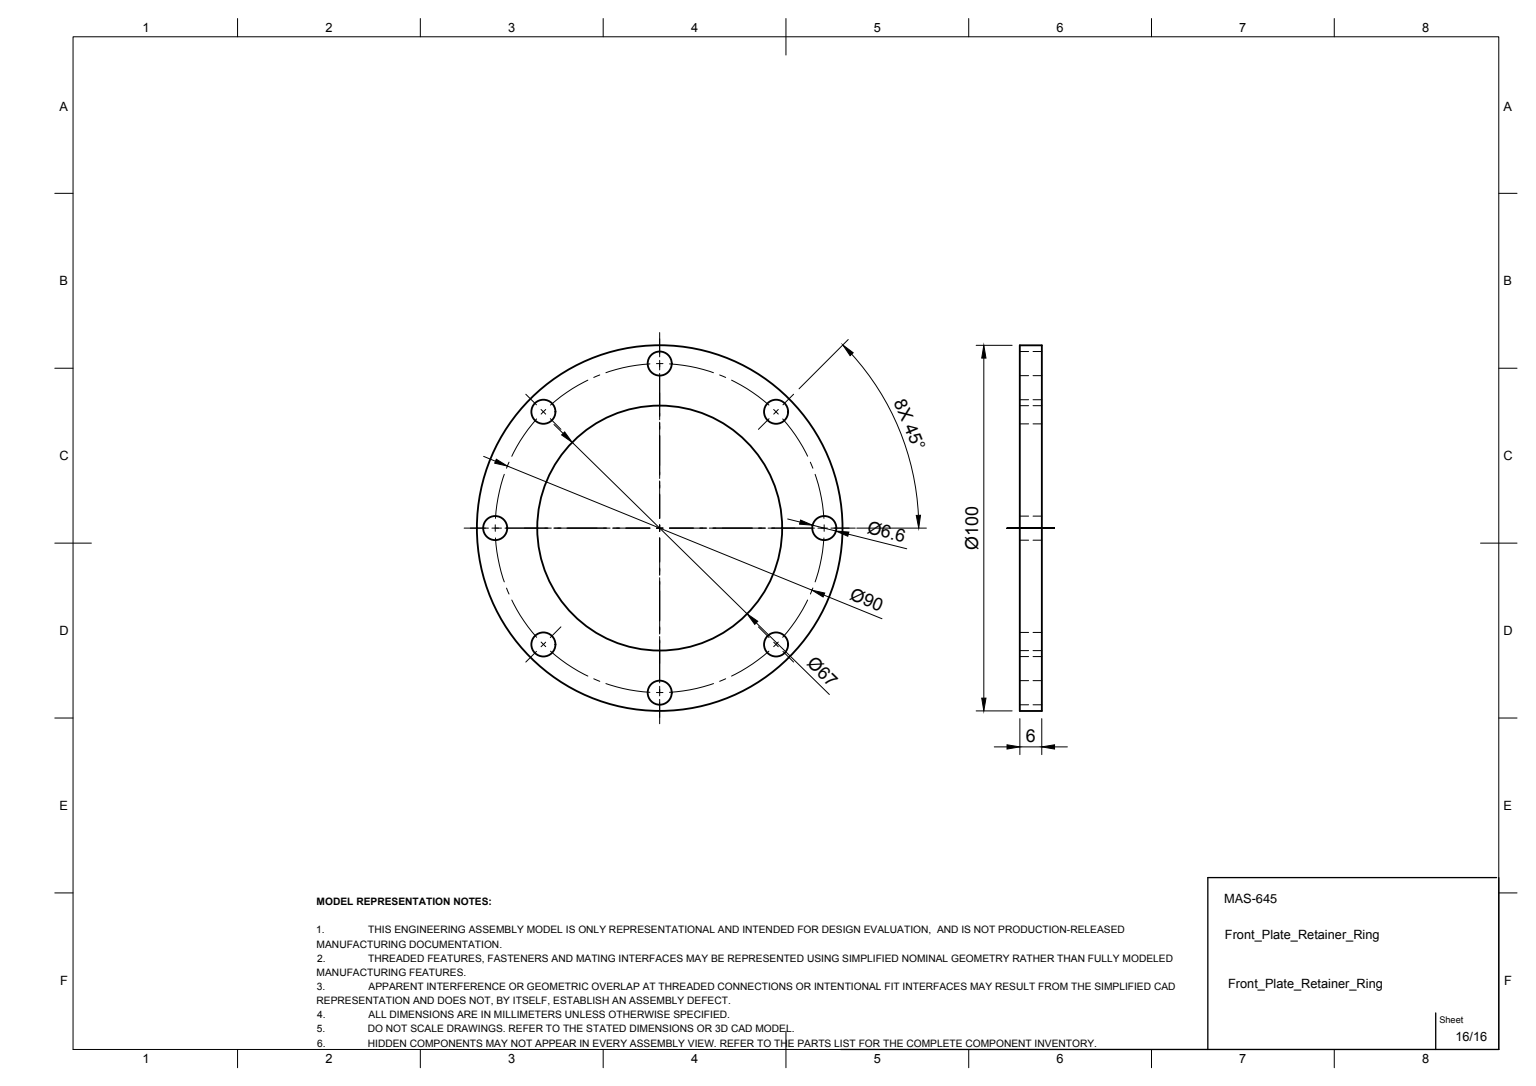
ISO-10303-21;
HEADER;
FILE_DESCRIPTION((''),'2;1');
FILE_NAME('Front_Plate_Retainer_Ring.step','2026-10-09T10:54:55-07:00',(''),(''),'','','');
FILE_SCHEMA (('AUTOMOTIVE_DESIGN { 1 0 10303 214 3 1 1 }'));
ENDSEC;
DATA;
#10=MECHANICAL_DESIGN_GEOMETRIC_PRESENTATION_REPRESENTATION('',(#609),#63824);
#579=SHAPE_REPRESENTATION_RELATIONSHIP('SRR','None',#63893,#594) ;
#594=ADVANCED_BREP_SHAPE_REPRESENTATION('',(#624),#63823) ;
#609=STYLED_ITEM('',(#63963),#624) ;
#624=MANIFOLD_SOLID_BREP('Body1',#15508) ;
#814=FACE_BOUND('',#3455,.T.) ;
#815=FACE_BOUND('',#3456,.T.) ;
#816=FACE_BOUND('',#3457,.T.) ;
#817=FACE_BOUND('',#3458,.T.) ;
#818=FACE_BOUND('',#3459,.T.) ;
#819=FACE_BOUND('',#3460,.T.) ;
#820=FACE_BOUND('',#3461,.T.) ;
#821=FACE_BOUND('',#3462,.T.) ;
#822=FACE_BOUND('',#3463,.T.) ;
#823=FACE_BOUND('',#3465,.T.) ;
#824=FACE_BOUND('',#3466,.T.) ;
#825=FACE_BOUND('',#3467,.T.) ;
#826=FACE_BOUND('',#3468,.T.) ;
#827=FACE_BOUND('',#3469,.T.) ;
#828=FACE_BOUND('',#3470,.T.) ;
#829=FACE_BOUND('',#3471,.T.) ;
#830=FACE_BOUND('',#3472,.T.) ;
#831=FACE_BOUND('',#3473,.T.) ;
#1114=PLANE('',#17883) ;
#1115=PLANE('',#17884) ;
#1535=CYLINDRICAL_SURFACE('',#17853,3.3) ;
#1536=CYLINDRICAL_SURFACE('',#17856,3.3) ;
#1537=CYLINDRICAL_SURFACE('',#17859,3.3) ;
#1538=CYLINDRICAL_SURFACE('',#17862,3.3) ;
#1539=CYLINDRICAL_SURFACE('',#17865,3.3) ;
#1540=CYLINDRICAL_SURFACE('',#17868,3.3) ;
#1541=CYLINDRICAL_SURFACE('',#17871,3.3) ;
#1542=CYLINDRICAL_SURFACE('',#17874,3.3) ;
#1543=CYLINDRICAL_SURFACE('',#17877,33.5) ;
#1544=CYLINDRICAL_SURFACE('',#17880,50.) ;
#2394=FACE_OUTER_BOUND('',#3444,.T.) ;
#2395=FACE_OUTER_BOUND('',#3445,.T.) ;
#2396=FACE_OUTER_BOUND('',#3446,.T.) ;
#2397=FACE_OUTER_BOUND('',#3447,.T.) ;
#2398=FACE_OUTER_BOUND('',#3448,.T.) ;
#2399=FACE_OUTER_BOUND('',#3449,.T.) ;
#2400=FACE_OUTER_BOUND('',#3450,.T.) ;
#2401=FACE_OUTER_BOUND('',#3451,.T.) ;
#2402=FACE_OUTER_BOUND('',#3452,.T.) ;
#2403=FACE_OUTER_BOUND('',#3453,.T.) ;
#2404=FACE_OUTER_BOUND('',#3454,.T.) ;
#2405=FACE_OUTER_BOUND('',#3464,.T.) ;
#3444=EDGE_LOOP('',(#14436,#14437,#14438,#14439)) ;
#3445=EDGE_LOOP('',(#14440,#14441,#14442,#14443)) ;
#3446=EDGE_LOOP('',(#14444,#14445,#14446,#14447)) ;
#3447=EDGE_LOOP('',(#14448,#14449,#14450,#14451)) ;
#3448=EDGE_LOOP('',(#14452,#14453,#14454,#14455)) ;
#3449=EDGE_LOOP('',(#14456,#14457,#14458,#14459)) ;
#3450=EDGE_LOOP('',(#14460,#14461,#14462,#14463)) ;
#3451=EDGE_LOOP('',(#14464,#14465,#14466,#14467)) ;
#3452=EDGE_LOOP('',(#14468,#14469,#14470,#14471)) ;
#3453=EDGE_LOOP('',(#14472,#14473,#14474,#14475)) ;
#3454=EDGE_LOOP('',(#14476)) ;
#3455=EDGE_LOOP('',(#14477)) ;
#3456=EDGE_LOOP('',(#14478)) ;
#3457=EDGE_LOOP('',(#14479)) ;
#3458=EDGE_LOOP('',(#14480)) ;
#3459=EDGE_LOOP('',(#14481)) ;
#3460=EDGE_LOOP('',(#14482)) ;
#3461=EDGE_LOOP('',(#14483)) ;
#3462=EDGE_LOOP('',(#14484)) ;
#3463=EDGE_LOOP('',(#14485)) ;
#3464=EDGE_LOOP('',(#14486)) ;
#3465=EDGE_LOOP('',(#14487)) ;
#3466=EDGE_LOOP('',(#14488)) ;
#3467=EDGE_LOOP('',(#14489)) ;
#3468=EDGE_LOOP('',(#14490)) ;
#3469=EDGE_LOOP('',(#14491)) ;
#3470=EDGE_LOOP('',(#14492)) ;
#3471=EDGE_LOOP('',(#14493)) ;
#3472=EDGE_LOOP('',(#14494)) ;
#3473=EDGE_LOOP('',(#14495)) ;
#4670=CIRCLE('',#17854,3.3) ;
#4671=CIRCLE('',#17855,3.3) ;
#4672=CIRCLE('',#17857,3.3) ;
#4673=CIRCLE('',#17858,3.3) ;
#4674=CIRCLE('',#17860,3.3) ;
#4675=CIRCLE('',#17861,3.3) ;
#4676=CIRCLE('',#17863,3.3) ;
#4677=CIRCLE('',#17864,3.3) ;
#4678=CIRCLE('',#17866,3.3) ;
#4679=CIRCLE('',#17867,3.3) ;
#4680=CIRCLE('',#17869,3.3) ;
#4681=CIRCLE('',#17870,3.3) ;
#4682=CIRCLE('',#17872,3.3) ;
#4683=CIRCLE('',#17873,3.3) ;
#4684=CIRCLE('',#17875,3.3) ;
#4685=CIRCLE('',#17876,3.3) ;
#4686=CIRCLE('',#17878,33.5) ;
#4687=CIRCLE('',#17879,33.5) ;
#4688=CIRCLE('',#17881,50.) ;
#4689=CIRCLE('',#17882,50.) ;
#5336=LINE('',#63716,#5992) ;
#5337=LINE('',#63722,#5993) ;
#5338=LINE('',#63728,#5994) ;
#5339=LINE('',#63734,#5995) ;
#5340=LINE('',#63740,#5996) ;
#5341=LINE('',#63746,#5997) ;
#5342=LINE('',#63752,#5998) ;
#5343=LINE('',#63758,#5999) ;
#5344=LINE('',#63764,#6000) ;
#5345=LINE('',#63770,#6001) ;
#5992=VECTOR('',#22908,3.3) ;
#5993=VECTOR('',#22915,3.3) ;
#5994=VECTOR('',#22922,3.3) ;
#5995=VECTOR('',#22929,3.3) ;
#5996=VECTOR('',#22936,3.3) ;
#5997=VECTOR('',#22943,3.3) ;
#5998=VECTOR('',#22950,3.3) ;
#5999=VECTOR('',#22957,3.3) ;
#6000=VECTOR('',#22964,33.5) ;
#6001=VECTOR('',#22971,50.) ;
#7435=VERTEX_POINT('',#63713) ;
#7436=VERTEX_POINT('',#63715) ;
#7437=VERTEX_POINT('',#63719) ;
#7438=VERTEX_POINT('',#63721) ;
#7439=VERTEX_POINT('',#63725) ;
#7440=VERTEX_POINT('',#63727) ;
#7441=VERTEX_POINT('',#63731) ;
#7442=VERTEX_POINT('',#63733) ;
#7443=VERTEX_POINT('',#63737) ;
#7444=VERTEX_POINT('',#63739) ;
#7445=VERTEX_POINT('',#63743) ;
#7446=VERTEX_POINT('',#63745) ;
#7447=VERTEX_POINT('',#63749) ;
#7448=VERTEX_POINT('',#63751) ;
#7449=VERTEX_POINT('',#63755) ;
#7450=VERTEX_POINT('',#63757) ;
#7451=VERTEX_POINT('',#63761) ;
#7452=VERTEX_POINT('',#63763) ;
#7453=VERTEX_POINT('',#63767) ;
#7454=VERTEX_POINT('',#63769) ;
#9772=EDGE_CURVE('',#7435,#7435,#4670,.T.) ;
#9773=EDGE_CURVE('',#7435,#7436,#5336,.T.) ;
#9774=EDGE_CURVE('',#7436,#7436,#4671,.T.) ;
#9775=EDGE_CURVE('',#7437,#7437,#4672,.T.) ;
#9776=EDGE_CURVE('',#7437,#7438,#5337,.T.) ;
#9777=EDGE_CURVE('',#7438,#7438,#4673,.T.) ;
#9778=EDGE_CURVE('',#7439,#7439,#4674,.T.) ;
#9779=EDGE_CURVE('',#7439,#7440,#5338,.T.) ;
#9780=EDGE_CURVE('',#7440,#7440,#4675,.T.) ;
#9781=EDGE_CURVE('',#7441,#7441,#4676,.T.) ;
#9782=EDGE_CURVE('',#7441,#7442,#5339,.T.) ;
#9783=EDGE_CURVE('',#7442,#7442,#4677,.T.) ;
#9784=EDGE_CURVE('',#7443,#7443,#4678,.T.) ;
#9785=EDGE_CURVE('',#7443,#7444,#5340,.T.) ;
#9786=EDGE_CURVE('',#7444,#7444,#4679,.T.) ;
#9787=EDGE_CURVE('',#7445,#7445,#4680,.T.) ;
#9788=EDGE_CURVE('',#7445,#7446,#5341,.T.) ;
#9789=EDGE_CURVE('',#7446,#7446,#4681,.T.) ;
#9790=EDGE_CURVE('',#7447,#7447,#4682,.T.) ;
#9791=EDGE_CURVE('',#7447,#7448,#5342,.T.) ;
#9792=EDGE_CURVE('',#7448,#7448,#4683,.T.) ;
#9793=EDGE_CURVE('',#7449,#7449,#4684,.T.) ;
#9794=EDGE_CURVE('',#7449,#7450,#5343,.T.) ;
#9795=EDGE_CURVE('',#7450,#7450,#4685,.T.) ;
#9796=EDGE_CURVE('',#7451,#7451,#4686,.T.) ;
#9797=EDGE_CURVE('',#7451,#7452,#5344,.T.) ;
#9798=EDGE_CURVE('',#7452,#7452,#4687,.T.) ;
#9799=EDGE_CURVE('',#7453,#7453,#4688,.T.) ;
#9800=EDGE_CURVE('',#7453,#7454,#5345,.T.) ;
#9801=EDGE_CURVE('',#7454,#7454,#4689,.T.) ;
#14436=ORIENTED_EDGE('',*,*,#9772,.T.) ;
#14437=ORIENTED_EDGE('',*,*,#9773,.T.) ;
#14438=ORIENTED_EDGE('',*,*,#9774,.T.) ;
#14439=ORIENTED_EDGE('',*,*,#9773,.F.) ;
#14440=ORIENTED_EDGE('',*,*,#9775,.T.) ;
#14441=ORIENTED_EDGE('',*,*,#9776,.T.) ;
#14442=ORIENTED_EDGE('',*,*,#9777,.T.) ;
#14443=ORIENTED_EDGE('',*,*,#9776,.F.) ;
#14444=ORIENTED_EDGE('',*,*,#9778,.T.) ;
#14445=ORIENTED_EDGE('',*,*,#9779,.T.) ;
#14446=ORIENTED_EDGE('',*,*,#9780,.T.) ;
#14447=ORIENTED_EDGE('',*,*,#9779,.F.) ;
#14448=ORIENTED_EDGE('',*,*,#9781,.T.) ;
#14449=ORIENTED_EDGE('',*,*,#9782,.T.) ;
#14450=ORIENTED_EDGE('',*,*,#9783,.T.) ;
#14451=ORIENTED_EDGE('',*,*,#9782,.F.) ;
#14452=ORIENTED_EDGE('',*,*,#9784,.T.) ;
#14453=ORIENTED_EDGE('',*,*,#9785,.T.) ;
#14454=ORIENTED_EDGE('',*,*,#9786,.T.) ;
#14455=ORIENTED_EDGE('',*,*,#9785,.F.) ;
#14456=ORIENTED_EDGE('',*,*,#9787,.T.) ;
#14457=ORIENTED_EDGE('',*,*,#9788,.T.) ;
#14458=ORIENTED_EDGE('',*,*,#9789,.T.) ;
#14459=ORIENTED_EDGE('',*,*,#9788,.F.) ;
#14460=ORIENTED_EDGE('',*,*,#9790,.T.) ;
#14461=ORIENTED_EDGE('',*,*,#9791,.T.) ;
#14462=ORIENTED_EDGE('',*,*,#9792,.T.) ;
#14463=ORIENTED_EDGE('',*,*,#9791,.F.) ;
#14464=ORIENTED_EDGE('',*,*,#9793,.T.) ;
#14465=ORIENTED_EDGE('',*,*,#9794,.T.) ;
#14466=ORIENTED_EDGE('',*,*,#9795,.T.) ;
#14467=ORIENTED_EDGE('',*,*,#9794,.F.) ;
#14468=ORIENTED_EDGE('',*,*,#9796,.T.) ;
#14469=ORIENTED_EDGE('',*,*,#9797,.T.) ;
#14470=ORIENTED_EDGE('',*,*,#9798,.T.) ;
#14471=ORIENTED_EDGE('',*,*,#9797,.F.) ;
#14472=ORIENTED_EDGE('',*,*,#9799,.T.) ;
#14473=ORIENTED_EDGE('',*,*,#9800,.T.) ;
#14474=ORIENTED_EDGE('',*,*,#9801,.T.) ;
#14475=ORIENTED_EDGE('',*,*,#9800,.F.) ;
#14476=ORIENTED_EDGE('',*,*,#9799,.F.) ;
#14477=ORIENTED_EDGE('',*,*,#9772,.F.) ;
#14478=ORIENTED_EDGE('',*,*,#9775,.F.) ;
#14479=ORIENTED_EDGE('',*,*,#9778,.F.) ;
#14480=ORIENTED_EDGE('',*,*,#9781,.F.) ;
#14481=ORIENTED_EDGE('',*,*,#9784,.F.) ;
#14482=ORIENTED_EDGE('',*,*,#9787,.F.) ;
#14483=ORIENTED_EDGE('',*,*,#9790,.F.) ;
#14484=ORIENTED_EDGE('',*,*,#9793,.F.) ;
#14485=ORIENTED_EDGE('',*,*,#9798,.F.) ;
#14486=ORIENTED_EDGE('',*,*,#9801,.F.) ;
#14487=ORIENTED_EDGE('',*,*,#9774,.F.) ;
#14488=ORIENTED_EDGE('',*,*,#9777,.F.) ;
#14489=ORIENTED_EDGE('',*,*,#9780,.F.) ;
#14490=ORIENTED_EDGE('',*,*,#9783,.F.) ;
#14491=ORIENTED_EDGE('',*,*,#9786,.F.) ;
#14492=ORIENTED_EDGE('',*,*,#9789,.F.) ;
#14493=ORIENTED_EDGE('',*,*,#9792,.F.) ;
#14494=ORIENTED_EDGE('',*,*,#9795,.F.) ;
#14495=ORIENTED_EDGE('',*,*,#9796,.F.) ;
#15482=ADVANCED_FACE('',(#2394),#1535,.F.) ;
#15483=ADVANCED_FACE('',(#2395),#1536,.F.) ;
#15484=ADVANCED_FACE('',(#2396),#1537,.F.) ;
#15485=ADVANCED_FACE('',(#2397),#1538,.F.) ;
#15486=ADVANCED_FACE('',(#2398),#1539,.F.) ;
#15487=ADVANCED_FACE('',(#2399),#1540,.F.) ;
#15488=ADVANCED_FACE('',(#2400),#1541,.F.) ;
#15489=ADVANCED_FACE('',(#2401),#1542,.F.) ;
#15490=ADVANCED_FACE('',(#2402),#1543,.F.) ;
#15491=ADVANCED_FACE('',(#2403),#1544,.T.) ;
#15492=ADVANCED_FACE('',(#2404,#814,#815,#816,#817,#818,#819,#820,#821,
#822),#1114,.T.) ;
#15493=ADVANCED_FACE('',(#2405,#823,#824,#825,#826,#827,#828,#829,#830,
#831),#1115,.F.) ;
#15508=CLOSED_SHELL('',(#15482,#15483,#15484,#15485,#15486,#15487,#15488,
#15489,#15490,#15491,#15492,#15493)) ;
#17852=AXIS2_PLACEMENT_3D('',#63711,#22902,#22903) ;
#17853=AXIS2_PLACEMENT_3D('',#63712,#22904,#22905) ;
#17854=AXIS2_PLACEMENT_3D('',#63714,#22906,#22907) ;
#17855=AXIS2_PLACEMENT_3D('',#63717,#22909,#22910) ;
#17856=AXIS2_PLACEMENT_3D('',#63718,#22911,#22912) ;
#17857=AXIS2_PLACEMENT_3D('',#63720,#22913,#22914) ;
#17858=AXIS2_PLACEMENT_3D('',#63723,#22916,#22917) ;
#17859=AXIS2_PLACEMENT_3D('',#63724,#22918,#22919) ;
#17860=AXIS2_PLACEMENT_3D('',#63726,#22920,#22921) ;
#17861=AXIS2_PLACEMENT_3D('',#63729,#22923,#22924) ;
#17862=AXIS2_PLACEMENT_3D('',#63730,#22925,#22926) ;
#17863=AXIS2_PLACEMENT_3D('',#63732,#22927,#22928) ;
#17864=AXIS2_PLACEMENT_3D('',#63735,#22930,#22931) ;
#17865=AXIS2_PLACEMENT_3D('',#63736,#22932,#22933) ;
#17866=AXIS2_PLACEMENT_3D('',#63738,#22934,#22935) ;
#17867=AXIS2_PLACEMENT_3D('',#63741,#22937,#22938) ;
#17868=AXIS2_PLACEMENT_3D('',#63742,#22939,#22940) ;
#17869=AXIS2_PLACEMENT_3D('',#63744,#22941,#22942) ;
#17870=AXIS2_PLACEMENT_3D('',#63747,#22944,#22945) ;
#17871=AXIS2_PLACEMENT_3D('',#63748,#22946,#22947) ;
#17872=AXIS2_PLACEMENT_3D('',#63750,#22948,#22949) ;
#17873=AXIS2_PLACEMENT_3D('',#63753,#22951,#22952) ;
#17874=AXIS2_PLACEMENT_3D('',#63754,#22953,#22954) ;
#17875=AXIS2_PLACEMENT_3D('',#63756,#22955,#22956) ;
#17876=AXIS2_PLACEMENT_3D('',#63759,#22958,#22959) ;
#17877=AXIS2_PLACEMENT_3D('',#63760,#22960,#22961) ;
#17878=AXIS2_PLACEMENT_3D('',#63762,#22962,#22963) ;
#17879=AXIS2_PLACEMENT_3D('',#63765,#22965,#22966) ;
#17880=AXIS2_PLACEMENT_3D('',#63766,#22967,#22968) ;
#17881=AXIS2_PLACEMENT_3D('',#63768,#22969,#22970) ;
#17882=AXIS2_PLACEMENT_3D('',#63771,#22972,#22973) ;
#17883=AXIS2_PLACEMENT_3D('',#63772,#22974,#22975) ;
#17884=AXIS2_PLACEMENT_3D('',#63773,#22976,#22977) ;
#22902=DIRECTION('axis',(0.,0.,1.)) ;
#22903=DIRECTION('refdir',(1.,0.,0.)) ;
#22904=DIRECTION('center_axis',(2.46519032881566E-32,-1.97215226305253E-31,
1.)) ;
#22905=DIRECTION('ref_axis',(-1.,1.15088063745374E-32,2.46519032881566E-32)) ;
#22906=DIRECTION('center_axis',(-2.46519032881566E-32,1.97215226305253E-31,
-1.)) ;
#22907=DIRECTION('ref_axis',(-1.,1.15088063745374E-32,2.46519032881566E-32)) ;
#22908=DIRECTION('',(2.46519032881566E-32,-1.97215226305253E-31,1.)) ;
#22909=DIRECTION('center_axis',(2.46519032881566E-32,-1.97215226305253E-31,
1.)) ;
#22910=DIRECTION('ref_axis',(-1.,1.15088063745374E-32,2.46519032881566E-32)) ;
#22911=DIRECTION('center_axis',(2.46519032881566E-32,-1.97215226305253E-31,
1.)) ;
#22912=DIRECTION('ref_axis',(-1.,1.15088063745374E-32,2.46519032881566E-32)) ;
#22913=DIRECTION('center_axis',(-2.46519032881566E-32,1.97215226305253E-31,
-1.)) ;
#22914=DIRECTION('ref_axis',(-1.,1.15088063745374E-32,2.46519032881566E-32)) ;
#22915=DIRECTION('',(2.46519032881566E-32,-1.97215226305253E-31,1.)) ;
#22916=DIRECTION('center_axis',(2.46519032881566E-32,-1.97215226305253E-31,
1.)) ;
#22917=DIRECTION('ref_axis',(-1.,1.15088063745374E-32,2.46519032881566E-32)) ;
#22918=DIRECTION('center_axis',(2.46519032881566E-32,-1.97215226305253E-31,
1.)) ;
#22919=DIRECTION('ref_axis',(-1.,1.15088063745374E-32,2.46519032881566E-32)) ;
#22920=DIRECTION('center_axis',(-2.46519032881566E-32,1.97215226305253E-31,
-1.)) ;
#22921=DIRECTION('ref_axis',(-1.,1.15088063745374E-32,2.46519032881566E-32)) ;
#22922=DIRECTION('',(2.46519032881566E-32,-1.97215226305253E-31,1.)) ;
#22923=DIRECTION('center_axis',(2.46519032881566E-32,-1.97215226305253E-31,
1.)) ;
#22924=DIRECTION('ref_axis',(-1.,1.15088063745374E-32,2.46519032881566E-32)) ;
#22925=DIRECTION('center_axis',(2.46519032881566E-32,-1.97215226305253E-31,
1.)) ;
#22926=DIRECTION('ref_axis',(-1.,1.15088063745374E-32,2.46519032881566E-32)) ;
#22927=DIRECTION('center_axis',(-2.46519032881566E-32,1.97215226305253E-31,
-1.)) ;
#22928=DIRECTION('ref_axis',(-1.,1.15088063745374E-32,2.46519032881566E-32)) ;
#22929=DIRECTION('',(2.46519032881566E-32,-1.97215226305253E-31,1.)) ;
#22930=DIRECTION('center_axis',(2.46519032881566E-32,-1.97215226305253E-31,
1.)) ;
#22931=DIRECTION('ref_axis',(-1.,1.15088063745374E-32,2.46519032881566E-32)) ;
#22932=DIRECTION('center_axis',(2.46519032881566E-32,-1.97215226305253E-31,
1.)) ;
#22933=DIRECTION('ref_axis',(-1.,1.15088063745374E-32,2.46519032881566E-32)) ;
#22934=DIRECTION('center_axis',(-2.46519032881566E-32,1.97215226305253E-31,
-1.)) ;
#22935=DIRECTION('ref_axis',(-1.,1.15088063745374E-32,2.46519032881566E-32)) ;
#22936=DIRECTION('',(2.46519032881566E-32,-1.97215226305253E-31,1.)) ;
#22937=DIRECTION('center_axis',(2.46519032881566E-32,-1.97215226305253E-31,
1.)) ;
#22938=DIRECTION('ref_axis',(-1.,1.15088063745374E-32,2.46519032881566E-32)) ;
#22939=DIRECTION('center_axis',(2.46519032881566E-32,-1.97215226305253E-31,
1.)) ;
#22940=DIRECTION('ref_axis',(-1.,1.15088063745374E-32,2.46519032881566E-32)) ;
#22941=DIRECTION('center_axis',(-2.46519032881566E-32,1.97215226305253E-31,
-1.)) ;
#22942=DIRECTION('ref_axis',(-1.,1.15088063745374E-32,2.46519032881566E-32)) ;
#22943=DIRECTION('',(2.46519032881566E-32,-1.97215226305253E-31,1.)) ;
#22944=DIRECTION('center_axis',(2.46519032881566E-32,-1.97215226305253E-31,
1.)) ;
#22945=DIRECTION('ref_axis',(-1.,1.15088063745374E-32,2.46519032881566E-32)) ;
#22946=DIRECTION('center_axis',(2.46519032881566E-32,-1.97215226305253E-31,
1.)) ;
#22947=DIRECTION('ref_axis',(-1.,1.15088063745374E-32,2.46519032881566E-32)) ;
#22948=DIRECTION('center_axis',(-2.46519032881566E-32,1.97215226305253E-31,
-1.)) ;
#22949=DIRECTION('ref_axis',(-1.,1.15088063745374E-32,2.46519032881566E-32)) ;
#22950=DIRECTION('',(2.46519032881566E-32,-1.97215226305253E-31,1.)) ;
#22951=DIRECTION('center_axis',(2.46519032881566E-32,-1.97215226305253E-31,
1.)) ;
#22952=DIRECTION('ref_axis',(-1.,1.15088063745374E-32,2.46519032881566E-32)) ;
#22953=DIRECTION('center_axis',(2.46519032881566E-32,-1.97215226305253E-31,
1.)) ;
#22954=DIRECTION('ref_axis',(-1.,1.15088063745374E-32,2.46519032881566E-32)) ;
#22955=DIRECTION('center_axis',(-2.46519032881566E-32,1.97215226305253E-31,
-1.)) ;
#22956=DIRECTION('ref_axis',(-1.,1.15088063745374E-32,2.46519032881566E-32)) ;
#22957=DIRECTION('',(2.46519032881566E-32,-1.97215226305253E-31,1.)) ;
#22958=DIRECTION('center_axis',(2.46519032881566E-32,-1.97215226305253E-31,
1.)) ;
#22959=DIRECTION('ref_axis',(-1.,1.15088063745374E-32,2.46519032881566E-32)) ;
#22960=DIRECTION('center_axis',(-2.46519032881566E-32,1.97215226305253E-31,
-1.)) ;
#22961=DIRECTION('ref_axis',(1.,-1.15088063745374E-32,-2.46519032881566E-32)) ;
#22962=DIRECTION('center_axis',(2.46519032881566E-32,-1.97215226305253E-31,
1.)) ;
#22963=DIRECTION('ref_axis',(1.,-1.15088063745374E-32,-2.46519032881566E-32)) ;
#22964=DIRECTION('',(-2.46519032881566E-32,1.97215226305253E-31,-1.)) ;
#22965=DIRECTION('center_axis',(-2.46519032881566E-32,1.97215226305253E-31,
-1.)) ;
#22966=DIRECTION('ref_axis',(1.,-1.15088063745374E-32,-2.46519032881566E-32)) ;
#22967=DIRECTION('center_axis',(-2.46519032881566E-32,1.97215226305253E-31,
-1.)) ;
#22968=DIRECTION('ref_axis',(1.,-1.15088063745374E-32,-2.46519032881566E-32)) ;
#22969=DIRECTION('center_axis',(2.46519032881566E-32,-1.97215226305253E-31,
1.)) ;
#22970=DIRECTION('ref_axis',(1.,-1.15088063745374E-32,-2.46519032881566E-32)) ;
#22971=DIRECTION('',(2.46519032881566E-32,-1.97215226305253E-31,1.)) ;
#22972=DIRECTION('center_axis',(-2.46519032881566E-32,1.97215226305253E-31,
-1.)) ;
#22973=DIRECTION('ref_axis',(1.,-1.15088063745374E-32,-2.46519032881566E-32)) ;
#22974=DIRECTION('center_axis',(-2.46519032881566E-32,1.97215226305253E-31,
-1.)) ;
#22975=DIRECTION('ref_axis',(-1.,1.15088063745374E-32,2.46519032881566E-32)) ;
#22976=DIRECTION('center_axis',(-2.46519032881566E-32,1.97215226305253E-31,
-1.)) ;
#22977=DIRECTION('ref_axis',(-1.,1.15088063745374E-32,2.46519032881566E-32)) ;
#63711=CARTESIAN_POINT('',(0.,0.,0.)) ;
#63712=CARTESIAN_POINT('Origin',(45.,354.45,-156.)) ;
#63713=CARTESIAN_POINT('',(48.3,354.45,-154.)) ;
#63714=CARTESIAN_POINT('Origin',(45.,354.45,-154.)) ;
#63715=CARTESIAN_POINT('',(48.3,354.45,-148.)) ;
#63716=CARTESIAN_POINT('',(48.3,354.45,-156.)) ;
#63717=CARTESIAN_POINT('Origin',(45.,354.45,-148.)) ;
#63718=CARTESIAN_POINT('Origin',(-5.51091059616308E-15,399.45,-156.)) ;
#63719=CARTESIAN_POINT('',(3.29999999999999,399.45,-154.)) ;
#63720=CARTESIAN_POINT('Origin',(-5.51091059616308E-15,399.45,-154.)) ;
#63721=CARTESIAN_POINT('',(3.29999999999999,399.45,-148.)) ;
#63722=CARTESIAN_POINT('',(3.29999999999999,399.45,-156.)) ;
#63723=CARTESIAN_POINT('Origin',(-5.51091059616308E-15,399.45,-148.)) ;
#63724=CARTESIAN_POINT('Origin',(-45.,354.45,-156.)) ;
#63725=CARTESIAN_POINT('',(-41.7,354.45,-154.)) ;
#63726=CARTESIAN_POINT('Origin',(-45.,354.45,-154.)) ;
#63727=CARTESIAN_POINT('',(-41.7,354.45,-148.)) ;
#63728=CARTESIAN_POINT('',(-41.7,354.45,-156.)) ;
#63729=CARTESIAN_POINT('Origin',(-45.,354.45,-148.)) ;
#63730=CARTESIAN_POINT('Origin',(4.10374200494004E-30,309.45,-156.)) ;
#63731=CARTESIAN_POINT('',(3.3,309.45,-154.)) ;
#63732=CARTESIAN_POINT('Origin',(4.15304581151636E-30,309.45,-154.)) ;
#63733=CARTESIAN_POINT('',(3.3,309.45,-148.)) ;
#63734=CARTESIAN_POINT('',(3.3,309.45,-156.)) ;
#63735=CARTESIAN_POINT('Origin',(4.3009572312453E-30,309.45,-148.)) ;
#63736=CARTESIAN_POINT('Origin',(-31.8198051533946,322.630194846605,-156.)) ;
#63737=CARTESIAN_POINT('',(-28.5198051533946,322.630194846605,-154.)) ;
#63738=CARTESIAN_POINT('Origin',(-31.8198051533946,322.630194846605,-154.)) ;
#63739=CARTESIAN_POINT('',(-28.5198051533946,322.630194846605,-148.)) ;
#63740=CARTESIAN_POINT('',(-28.5198051533946,322.630194846605,-156.)) ;
#63741=CARTESIAN_POINT('Origin',(-31.8198051533946,322.630194846605,-148.)) ;
#63742=CARTESIAN_POINT('Origin',(-31.8198051533946,386.269805153395,-156.)) ;
#63743=CARTESIAN_POINT('',(-28.5198051533946,386.269805153395,-154.)) ;
#63744=CARTESIAN_POINT('Origin',(-31.8198051533946,386.269805153395,-154.)) ;
#63745=CARTESIAN_POINT('',(-28.5198051533946,386.269805153395,-148.)) ;
#63746=CARTESIAN_POINT('',(-28.5198051533946,386.269805153395,-156.)) ;
#63747=CARTESIAN_POINT('Origin',(-31.8198051533946,386.269805153395,-148.)) ;
#63748=CARTESIAN_POINT('Origin',(31.8198051533946,386.269805153395,-156.)) ;
#63749=CARTESIAN_POINT('',(35.1198051533946,386.269805153395,-154.)) ;
#63750=CARTESIAN_POINT('Origin',(31.8198051533946,386.269805153395,-154.)) ;
#63751=CARTESIAN_POINT('',(35.1198051533946,386.269805153395,-148.)) ;
#63752=CARTESIAN_POINT('',(35.1198051533946,386.269805153395,-156.)) ;
#63753=CARTESIAN_POINT('Origin',(31.8198051533946,386.269805153395,-148.)) ;
#63754=CARTESIAN_POINT('Origin',(31.8198051533946,322.630194846605,-156.)) ;
#63755=CARTESIAN_POINT('',(35.1198051533946,322.630194846605,-154.)) ;
#63756=CARTESIAN_POINT('Origin',(31.8198051533946,322.630194846605,-154.)) ;
#63757=CARTESIAN_POINT('',(35.1198051533946,322.630194846605,-148.)) ;
#63758=CARTESIAN_POINT('',(35.1198051533946,322.630194846605,-156.)) ;
#63759=CARTESIAN_POINT('Origin',(31.8198051533946,322.630194846605,-148.)) ;
#63760=CARTESIAN_POINT('Origin',(4.67094209837054E-30,354.45,-154.)) ;
#63761=CARTESIAN_POINT('',(-33.5,354.45,-148.)) ;
#63762=CARTESIAN_POINT('Origin',(4.81885351809948E-30,354.45,-148.)) ;
#63763=CARTESIAN_POINT('',(-33.5,354.45,-154.)) ;
#63764=CARTESIAN_POINT('',(-33.5,354.45,-154.)) ;
#63765=CARTESIAN_POINT('Origin',(4.67094209837054E-30,354.45,-154.)) ;
#63766=CARTESIAN_POINT('Origin',(4.67094209837054E-30,354.45,-154.)) ;
#63767=CARTESIAN_POINT('',(-50.,354.45,-154.)) ;
#63768=CARTESIAN_POINT('Origin',(4.67094209837054E-30,354.45,-154.)) ;
#63769=CARTESIAN_POINT('',(-50.,354.45,-148.)) ;
#63770=CARTESIAN_POINT('',(-50.,354.45,-154.)) ;
#63771=CARTESIAN_POINT('Origin',(4.81885351809948E-30,354.45,-148.)) ;
#63772=CARTESIAN_POINT('Origin',(4.67094209837054E-30,354.45,-154.)) ;
#63773=CARTESIAN_POINT('Origin',(4.81885351809948E-30,354.45,-148.)) ;
#63806=UNCERTAINTY_MEASURE_WITH_UNIT(LENGTH_MEASURE(0.01),#63825,
'DISTANCE_ACCURACY_VALUE',
'Maximum model space distance between geometric entities at asserted c
onnectivities') ;
#63807=UNCERTAINTY_MEASURE_WITH_UNIT(LENGTH_MEASURE(0.01),#63825,
'DISTANCE_ACCURACY_VALUE',
'Maximum model space distance between geometric entities at asserted c
onnectivities') ;
#63823=(
GEOMETRIC_REPRESENTATION_CONTEXT(3)
GLOBAL_UNCERTAINTY_ASSIGNED_CONTEXT((#63806))
GLOBAL_UNIT_ASSIGNED_CONTEXT((#63825,#63827,#63828))
REPRESENTATION_CONTEXT('','3D')
) ;
#63824=(
GEOMETRIC_REPRESENTATION_CONTEXT(3)
GLOBAL_UNCERTAINTY_ASSIGNED_CONTEXT((#63807))
GLOBAL_UNIT_ASSIGNED_CONTEXT((#63825,#63827,#63828))
REPRESENTATION_CONTEXT('','3D')
) ;
#63825=(
LENGTH_UNIT()
NAMED_UNIT(*)
SI_UNIT(.MILLI.,.METRE.)
) ;
#63827=(
NAMED_UNIT(*)
PLANE_ANGLE_UNIT()
SI_UNIT($,.RADIAN.)
) ;
#63828=(
NAMED_UNIT(*)
SI_UNIT($,.STERADIAN.)
SOLID_ANGLE_UNIT()
) ;
#63844=SHAPE_DEFINITION_REPRESENTATION(#63860,#63893) ;
#63860=PRODUCT_DEFINITION_SHAPE('',$,#63910) ;
#63893=SHAPE_REPRESENTATION('',(#17852),#63823) ;
#63894=PRODUCT_DEFINITION_CONTEXT('part definition',#63944,'design') ;
#63910=PRODUCT_DEFINITION('Front_Plate_Retainer_Ring',
'Front_Plate_Retainer_Ring',#63926,#63894) ;
#63926=PRODUCT_DEFINITION_FORMATION('',$,#63961) ;
#63944=APPLICATION_CONTEXT(
'Core Data for Automotive Mechanical Design Process') ;
#63945=PRODUCT_CONTEXT('part definition',#63944,'mechanical') ;
#63961=PRODUCT('Front_Plate_Retainer_Ring','Front_Plate_Retainer_Ring',
$,(#63945)) ;
#63963=PRESENTATION_STYLE_ASSIGNMENT((#63968)) ;
#63968=SURFACE_STYLE_USAGE(.BOTH.,#63973) ;
#63973=SURFACE_SIDE_STYLE('',(#63978)) ;
#63978=SURFACE_STYLE_FILL_AREA(#63983) ;
#63983=FILL_AREA_STYLE('Opaque(160,160,160)',(#63988)) ;
#63988=FILL_AREA_STYLE_COLOUR('Opaque(160,160,160)',#63993) ;
#63993=COLOUR_RGB('Opaque(160,160,160)', 0.09019608, 0.27058824, 0.51372549) ;
ENDSEC;
END-ISO-10303-21;
